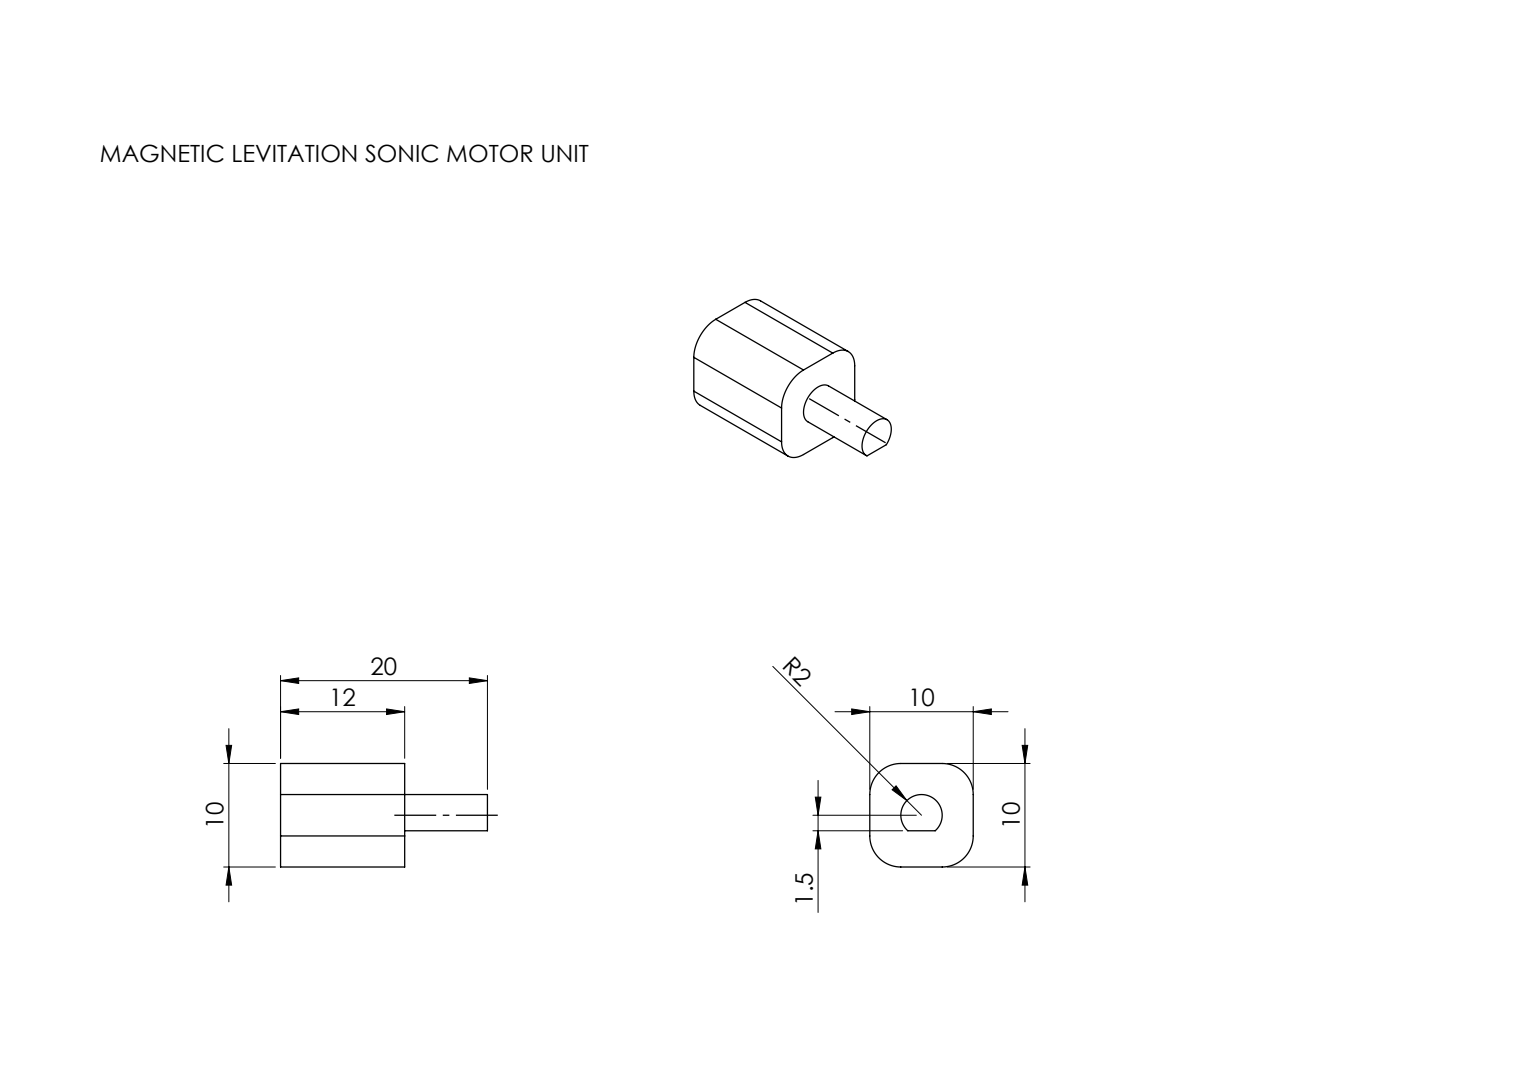
ISO-10303-21;
HEADER;
FILE_DESCRIPTION (('STEP AP214'),
    '1' );
FILE_NAME ('Magnetic Levitation Sonic Motor Unit.step',
    '2026-10-02T09:26:43',
    ( '' ),
    ( '' ),
    'SwSTEP 2.0',
    'SolidWorks 2026',
    '' );
FILE_SCHEMA (( 'AUTOMOTIVE_DESIGN' ));
ENDSEC;

DATA;
#65=DIRECTION ( 'NONE',  ( 1.000000000000000000, -0.000000000000000000, -0.000000000000000000 ) ) ;
#240=VERTEX_POINT ( 'NONE', #115266 ) ;
#450=CIRCLE ( 'NONE', #88369, 2.000000000000000000 ) ;
#508=ORIENTED_EDGE ( 'NONE', *, *, #3141, .T. ) ;
#1062=DIRECTION ( 'NONE',  ( -1.000000000000000000, 0.000000000000000000, 1.445602896647339656E-16 ) ) ;
#1136=ADVANCED_FACE ( 'NONE', ( #79104 ), #62037, .T. ) ;
#1254=CARTESIAN_POINT ( 'NONE',  ( 115.5000000000000000, 5.000000000000000000, -4.999999999999997335 ) ) ;
#1658=ORIENTED_EDGE ( 'NONE', *, *, #93470, .T. ) ;
#1663=ORIENTED_EDGE ( 'NONE', *, *, #28422, .T. ) ;
#1678=( GEOMETRIC_REPRESENTATION_CONTEXT ( 3 ) GLOBAL_UNCERTAINTY_ASSIGNED_CONTEXT ( ( #101904 ) ) GLOBAL_UNIT_ASSIGNED_CONTEXT ( ( #110801, #83298, #46567 ) ) REPRESENTATION_CONTEXT ( 'NONE', 'WORKASPACE' ) );
#1737=ORIENTED_EDGE ( 'NONE', *, *, #92849, .T. ) ;
#1889=VERTEX_POINT ( 'NONE', #49825 ) ;
#1942=AXIS2_PLACEMENT_3D ( 'NONE', #45673, #115030, #116960 ) ;
#2262=EDGE_CURVE ( 'NONE', #111941, #240, #82590, .T. ) ;
#2320=PRESENTATION_STYLE_ASSIGNMENT (( #29873 ) ) ;
#2577=DIRECTION ( 'NONE',  ( 0.000000000000000000, 0.000000000000000000, 1.000000000000000000 ) ) ;
#3141=EDGE_CURVE ( 'NONE', #1889, #72667, #15996, .T. ) ;
#3881=CARTESIAN_POINT ( 'NONE',  ( 127.5000000000000000, 2.000000000000000000, -1.999999999999998224 ) ) ;
#4111=ORIENTED_EDGE ( 'NONE', *, *, #2262, .T. ) ;
#4330=ORIENTED_EDGE ( 'NONE', *, *, #114609, .T. ) ;
#4691=SHAPE_REPRESENTATION_RELATIONSHIP ( 'NONE' , 'NONE' ,  #107120, #21197 ) ;
#5147=DIRECTION ( 'NONE',  ( 0.000000000000000000, 1.000000000000000000, -0.000000000000000000 ) ) ;
#6227=CARTESIAN_POINT ( 'NONE',  ( 115.5000000000000000, 2.000000000000000000, 5.000000000000003553 ) ) ;
#7736=ADVANCED_FACE ( 'NONE', ( #129346 ), #88749, .F. ) ;
#7761=DIRECTION ( 'NONE',  ( 7.228014483236698281E-17, 0.000000000000000000, 1.000000000000000000 ) ) ;
#8511=EDGE_CURVE ( 'NONE', #13812, #109878, #17393, .T. ) ;
#8802=CARTESIAN_POINT ( 'NONE',  ( 127.5000000000000000, -5.000000000000000000, -1.999999999999998224 ) ) ;
#9052=DIRECTION ( 'NONE',  ( -1.000000000000000000, 0.000000000000000000, 1.445602896647339656E-16 ) ) ;
#9433=ADVANCED_FACE ( 'NONE', ( #129511 ), #107901, .F. ) ;
#9447=AXIS2_PLACEMENT_3D ( 'NONE', #120852, #70463, #71758 ) ;
#10014=COLOUR_RGB ( '', 0.66274510, 0.83137255, 0.94901961) ;
#10439=AXIS2_PLACEMENT_3D ( 'NONE', #63271, #42355, #31888 ) ;
#10465=ORIENTED_EDGE ( 'NONE', *, *, #101781, .T. ) ;
#10644=CARTESIAN_POINT ( 'NONE',  ( 0.000000000000000000, 0.000000000000000000, 0.000000000000000000 ) ) ;
#10665=DIRECTION ( 'NONE',  ( 0.000000000000000000, 0.000000000000000000, -1.000000000000000000 ) ) ;
#11350=CARTESIAN_POINT ( 'NONE',  ( 127.5000000000000000, 5.000000000000000000, -4.999999999999998224 ) ) ;
#11517=SURFACE_STYLE_FILL_AREA ( #60003 ) ;
#11655=CARTESIAN_POINT ( 'NONE',  ( 127.5000000000000000, 2.000000000000000000, 5.000000000000001776 ) ) ;
#11783=CARTESIAN_POINT ( 'NONE',  ( 107.5000000000000142, 0.000000000000000000, 0.000000000000000000 ) ) ;
#12150=FILL_AREA_STYLE_COLOUR ( '', #52176 ) ;
#12190=EDGE_CURVE ( 'NONE', #36385, #240, #102708, .T. ) ;
#12224=CLOSED_SHELL ( 'NONE', ( #21549, #64318, #22970, #9433, #68328, #7736, #72582, #51956, #31701, #107579, #84007, #1136, #95844, #112044, #31528 ) ) ;
#12350=ORIENTED_EDGE ( 'NONE', *, *, #109024, .T. ) ;
#13249=ORIENTED_EDGE ( 'NONE', *, *, #43912, .F. ) ;
#13516=PLANE ( 'NONE',  #10439 ) ;
#13646=ORIENTED_EDGE ( 'NONE', *, *, #65383, .F. ) ;
#13812=VERTEX_POINT ( 'NONE', #6227 ) ;
#14010=CARTESIAN_POINT ( 'NONE',  ( 107.5000000000000142, -1.500000000000000222, -1.322875655532295136 ) ) ;
#14733=CYLINDRICAL_SURFACE ( 'NONE', #101479, 3.000000000000000000 ) ;
#14758=ORIENTED_EDGE ( 'NONE', *, *, #92576, .F. ) ;
#14831=ORIENTED_EDGE ( 'NONE', *, *, #41235, .T. ) ;
#15219=AXIS2_PLACEMENT_3D ( 'NONE', #88237, #19519, #9052 ) ;
#15562=CARTESIAN_POINT ( 'NONE',  ( 127.5000000000000000, -5.000000000000000000, -4.999999999999998224 ) ) ;
#15996=LINE ( 'NONE', #36954, #101692 ) ;
#16704=EDGE_LOOP ( 'NONE', ( #22045, #13249, #50877, #119234 ) ) ;
#16723=VERTEX_POINT ( 'NONE', #56935 ) ;
#16868=PLANE ( 'NONE',  #87019 ) ;
#16927=CARTESIAN_POINT ( 'NONE',  ( 115.5000000000000000, 0.000000000000000000, 0.000000000000000000 ) ) ;
#16966=EDGE_LOOP ( 'NONE', ( #102248, #67737, #34286, #98490 ) ) ;
#17271=DIRECTION ( 'NONE',  ( -1.000000000000000000, 0.000000000000000000, 7.228014483236698281E-17 ) ) ;
#17393=LINE ( 'NONE', #118836, #123704 ) ;
#17472=ORIENTED_EDGE ( 'NONE', *, *, #123464, .T. ) ;
#18382=CARTESIAN_POINT ( 'NONE',  ( 107.5000000000000142, 0.000000000000000000, 0.000000000000000000 ) ) ;
#18525=FACE_OUTER_BOUND ( 'NONE', #48553, .T. ) ;
#19100=PRODUCT_DEFINITION_FORMATION_WITH_SPECIFIED_SOURCE ( 'ANY', '', #126727, .NOT_KNOWN. ) ;
#19272=VECTOR ( 'NONE', #69817, 1000.000000000000000 ) ;
#19404=CYLINDRICAL_SURFACE ( 'NONE', #117385, 3.000000000000000000 ) ;
#19514=DIRECTION ( 'NONE',  ( -1.445602896647339656E-16, 0.000000000000000000, -1.000000000000000000 ) ) ;
#19519=DIRECTION ( 'NONE',  ( -1.445602896647339656E-16, 0.000000000000000000, -1.000000000000000000 ) ) ;
#20065=SURFACE_SIDE_STYLE ('',( #11517 ) ) ;
#20148=VERTEX_POINT ( 'NONE', #23352 ) ;
#20366=CYLINDRICAL_SURFACE ( 'NONE', #98432, 2.000000000000000000 ) ;
#20481=DIRECTION ( 'NONE',  ( 0.000000000000000000, 0.000000000000000000, -1.000000000000000000 ) ) ;
#20860=EDGE_CURVE ( 'NONE', #36385, #26275, #450, .T. ) ;
#21028=EDGE_CURVE ( 'NONE', #67896, #36385, #79981, .T. ) ;
#21197=ADVANCED_BREP_SHAPE_REPRESENTATION ( '', ( #100344, #108296 ), #1678 ) ;
#21549=ADVANCED_FACE ( 'NONE', ( #86151 ), #54142, .T. ) ;
#22045=ORIENTED_EDGE ( 'NONE', *, *, #39691, .T. ) ;
#22970=ADVANCED_FACE ( 'NONE', ( #100521, #58040 ), #29860, .F. ) ;
#23004=EDGE_LOOP ( 'NONE', ( #124572, #104293, #39056, #89225 ) ) ;
#23108=EDGE_LOOP ( 'NONE', ( #101575, #116612, #60474, #14758 ) ) ;
#23352=CARTESIAN_POINT ( 'NONE',  ( 127.5000000000000000, 2.000000000000000000, 5.000000000000001776 ) ) ;
#23547=AXIS2_PLACEMENT_3D ( 'NONE', #11783, #67297, #64749 ) ;
#23555=DIRECTION ( 'NONE',  ( 1.000000000000000000, 0.000000000000000000, -1.445602896647339656E-16 ) ) ;
#24253=VERTEX_POINT ( 'NONE', #107794 ) ;
#24764=AXIS2_PLACEMENT_3D ( 'NONE', #3881, #62817, #2577 ) ;
#24890=VECTOR ( 'NONE', #110517, 1000.000000000000000 ) ;
#25130=LINE ( 'NONE', #14010, #32508 ) ;
#25173=ORIENTED_EDGE ( 'NONE', *, *, #93470, .F. ) ;
#25217=ORIENTED_EDGE ( 'NONE', *, *, #65829, .F. ) ;
#25508=AXIS2_PLACEMENT_3D ( 'NONE', #64162, #104097, #82537 ) ;
#25638=FILL_AREA_STYLE_COLOUR ( '', #10014 ) ;
#25827=CARTESIAN_POINT ( 'NONE',  ( 0.000000000000000000, -5.000000000000000000, 0.000000000000000000 ) ) ;
#26275=VERTEX_POINT ( 'NONE', #82124 ) ;
#26426=DIRECTION ( 'NONE',  ( 0.000000000000000000, 0.000000000000000000, -1.000000000000000000 ) ) ;
#26535=EDGE_CURVE ( 'NONE', #13812, #82111, #34603, .T. ) ;
#26613=CARTESIAN_POINT ( 'NONE',  ( 107.5000000000000142, 0.000000000000000000, 0.000000000000000000 ) ) ;
#26943=( NAMED_UNIT ( * ) SI_UNIT ( $, .STERADIAN. ) SOLID_ANGLE_UNIT ( ) );
#28422=EDGE_CURVE ( 'NONE', #82111, #56575, #83767, .T. ) ;
#28472=DIRECTION ( 'NONE',  ( 1.000000000000000000, -0.000000000000000000, -7.228014483236698281E-17 ) ) ;
#28475=DIRECTION ( 'NONE',  ( 0.000000000000000000, 0.000000000000000000, 1.000000000000000000 ) ) ;
#29256=CARTESIAN_POINT ( 'NONE',  ( 127.5000000000000000, -2.000000000000000000, 2.000000000000001776 ) ) ;
#29359=CARTESIAN_POINT ( 'NONE',  ( 2.891205793294708895E-16, 2.000000000000000000, 2.000000000000020428 ) ) ;
#29454=AXIS2_PLACEMENT_3D ( 'NONE', #25827, #95859, #33710 ) ;
#29728=CIRCLE ( 'NONE', #25508, 2.000000000000000000 ) ;
#29854=EDGE_LOOP ( 'NONE', ( #1737, #1658, #71670, #1663 ) ) ;
#29860=PLANE ( 'NONE',  #101273 ) ;
#29873=SURFACE_STYLE_USAGE ( .BOTH. , #20065 ) ;
#29890=CARTESIAN_POINT ( 'NONE',  ( 127.5000000000000000, -2.000000000000000000, 5.000000000000001776 ) ) ;
#30716=EDGE_CURVE ( 'NONE', #127948, #48914, #48562, .T. ) ;
#30808=DIRECTION ( 'NONE',  ( 0.000000000000000000, 0.000000000000000000, 1.000000000000000000 ) ) ;
#31320=DIRECTION ( 'NONE',  ( -1.000000000000000000, -0.000000000000000000, 1.445602896647339656E-16 ) ) ;
#31425=AXIS2_PLACEMENT_3D ( 'NONE', #60506, #39589, #90580 ) ;
#31528=ADVANCED_FACE ( 'NONE', ( #36513 ), #76424, .T. ) ;
#31598=ORIENTED_EDGE ( 'NONE', *, *, #32466, .T. ) ;
#31701=ADVANCED_FACE ( 'NONE', ( #34426 ), #14733, .T. ) ;
#31888=DIRECTION ( 'NONE',  ( 0.000000000000000000, -0.000000000000000000, -1.000000000000000000 ) ) ;
#32125=CIRCLE ( 'NONE', #128264, 3.000000000000000000 ) ;
#32466=EDGE_CURVE ( 'NONE', #127948, #72667, #82415, .T. ) ;
#32508=VECTOR ( 'NONE', #36260, 1000.000000000000000 ) ;
#32961=ORIENTED_EDGE ( 'NONE', *, *, #35227, .T. ) ;
#33008=ORIENTED_EDGE ( 'NONE', *, *, #77146, .T. ) ;
#33110=STYLED_ITEM ( 'NONE', ( #74118 ), #21197 ) ;
#33710=DIRECTION ( 'NONE',  ( 0.000000000000000000, -0.000000000000000000, -1.000000000000000000 ) ) ;
#34286=ORIENTED_EDGE ( 'NONE', *, *, #109024, .F. ) ;
#34426=FACE_OUTER_BOUND ( 'NONE', #104073, .T. ) ;
#34603=CIRCLE ( 'NONE', #47193, 3.000000000000000000 ) ;
#35227=EDGE_CURVE ( 'NONE', #44931, #67896, #83560, .T. ) ;
#35416=CIRCLE ( 'NONE', #70923, 3.000000000000000000 ) ;
#35523=DIRECTION ( 'NONE',  ( 0.000000000000000000, 0.000000000000000000, 1.000000000000000000 ) ) ;
#35867=DIRECTION ( 'NONE',  ( -0.000000000000000000, -0.000000000000000000, -1.000000000000000000 ) ) ;
#35956=ORIENTED_EDGE ( 'NONE', *, *, #128508, .F. ) ;
#36260=DIRECTION ( 'NONE',  ( 1.000000000000000000, -0.000000000000000000, -0.000000000000000000 ) ) ;
#36385=VERTEX_POINT ( 'NONE', #110445 ) ;
#36513=FACE_OUTER_BOUND ( 'NONE', #102155, .T. ) ;
#36519=VECTOR ( 'NONE', #95962, 1000.000000000000000 ) ;
#36954=CARTESIAN_POINT ( 'NONE',  ( 115.5000000000000000, -2.000000000000000000, -4.999999999999997335 ) ) ;
#37326=ORIENTED_EDGE ( 'NONE', *, *, #77740, .T. ) ;
#37461=DIRECTION ( 'NONE',  ( 1.000000000000000000, -0.000000000000000000, -7.228014483236698281E-17 ) ) ;
#37515=MECHANICAL_DESIGN_GEOMETRIC_PRESENTATION_REPRESENTATION('',(#91884),#56365);
#38091=CARTESIAN_POINT ( 'NONE',  ( 115.5000000000000000, 0.000000000000000000, 0.000000000000000000 ) ) ;
#38139=VECTOR ( 'NONE', #23555, 1000.000000000000000 ) ;
#38261=FACE_OUTER_BOUND ( 'NONE', #73697, .T. ) ;
#38932=VERTEX_POINT ( 'NONE', #58490 ) ;
#39056=ORIENTED_EDGE ( 'NONE', *, *, #77146, .F. ) ;
#39564=ORIENTED_EDGE ( 'NONE', *, *, #128051, .F. ) ;
#39589=DIRECTION ( 'NONE',  ( -1.000000000000000000, 0.000000000000000000, 0.000000000000000000 ) ) ;
#39677=CARTESIAN_POINT ( 'NONE',  ( 127.5000000000000000, 5.000000000000000000, -4.999999999999998224 ) ) ;
#39691=EDGE_CURVE ( 'NONE', #84059, #111941, #77154, .T. ) ;
#39853=CIRCLE ( 'NONE', #31425, 2.000000000000000000 ) ;
#40530=EDGE_CURVE ( 'NONE', #66994, #47269, #55118, .T. ) ;
#40555=LINE ( 'NONE', #100100, #75993 ) ;
#40637=DIRECTION ( 'NONE',  ( -1.000000000000000000, 0.000000000000000000, 0.000000000000000000 ) ) ;
#40674=CARTESIAN_POINT ( 'NONE',  ( 107.5000000000000142, 0.000000000000000000, 0.000000000000000000 ) ) ;
#41021=LINE ( 'NONE', #29890, #19272 ) ;
#41235=EDGE_CURVE ( 'NONE', #20148, #13812, #62065, .T. ) ;
#41481=DIRECTION ( 'NONE',  ( -0.000000000000000000, -1.000000000000000000, -0.000000000000000000 ) ) ;
#41997=ORIENTED_EDGE ( 'NONE', *, *, #73950, .F. ) ;
#42355=DIRECTION ( 'NONE',  ( 0.000000000000000000, -1.000000000000000000, 0.000000000000000000 ) ) ;
#42949=AXIS2_PLACEMENT_3D ( 'NONE', #116083, #85335, #26426 ) ;
#43239=ORIENTED_EDGE ( 'NONE', *, *, #73950, .T. ) ;
#43912=EDGE_CURVE ( 'NONE', #67896, #111941, #129483, .T. ) ;
#44175=EDGE_LOOP ( 'NONE', ( #50268, #50582, #52858, #85813 ) ) ;
#44219=VERTEX_POINT ( 'NONE', #75668 ) ;
#44322=EDGE_LOOP ( 'NONE', ( #31598, #17472, #57035, #68258, #82847, #94300, #64121, #118110 ) ) ;
#44700=APPLICATION_CONTEXT ( 'automotive_design' ) ;
#44931=VERTEX_POINT ( 'NONE', #102724 ) ;
#45308=DIRECTION ( 'NONE',  ( 0.000000000000000000, 0.000000000000000000, 1.000000000000000000 ) ) ;
#45528=VECTOR ( 'NONE', #106603, 1000.000000000000000 ) ;
#45673=CARTESIAN_POINT ( 'NONE',  ( 115.5000000000000000, 2.000000000000000000, -1.999999999999997335 ) ) ;
#46357=CARTESIAN_POINT ( 'NONE',  ( 107.5000000000000142, -1.500000000000000222, -1.322875655532295136 ) ) ;
#46394=FACE_OUTER_BOUND ( 'NONE', #78387, .T. ) ;
#46567=( NAMED_UNIT ( * ) SI_UNIT ( $, .STERADIAN. ) SOLID_ANGLE_UNIT ( ) );
#47193=AXIS2_PLACEMENT_3D ( 'NONE', #51245, #58485, #20481 ) ;
#47269=VERTEX_POINT ( 'NONE', #98818 ) ;
#47614=ORIENTED_EDGE ( 'NONE', *, *, #88513, .T. ) ;
#47723=PRODUCT_CONTEXT ( 'NONE', #44700, 'mechanical' ) ;
#48220=CARTESIAN_POINT ( 'NONE',  ( 107.5000000000000142, -1.500000000000000222, 1.322875655532295136 ) ) ;
#48342=CARTESIAN_POINT ( 'NONE',  ( -1.445602896647332014E-16, 2.000000000000000000, -1.999999999999989120 ) ) ;
#48553=EDGE_LOOP ( 'NONE', ( #113735, #121629, #81596, #4111 ) ) ;
#48562=LINE ( 'NONE', #127758, #128709 ) ;
#48838=DIRECTION ( 'NONE',  ( 7.228014483236698281E-17, -0.000000000000000000, 1.000000000000000000 ) ) ;
#48914=VERTEX_POINT ( 'NONE', #62318 ) ;
#49825=CARTESIAN_POINT ( 'NONE',  ( 127.5000000000000000, -2.000000000000000000, -4.999999999999998224 ) ) ;
#50174=( NAMED_UNIT ( * ) SI_UNIT ( $, .STERADIAN. ) SOLID_ANGLE_UNIT ( ) );
#50268=ORIENTED_EDGE ( 'NONE', *, *, #20860, .F. ) ;
#50582=ORIENTED_EDGE ( 'NONE', *, *, #12190, .T. ) ;
#50877=ORIENTED_EDGE ( 'NONE', *, *, #35227, .F. ) ;
#51245=CARTESIAN_POINT ( 'NONE',  ( 115.5000000000000000, 2.000000000000000000, 2.000000000000003553 ) ) ;
#51462=( NAMED_UNIT ( * ) PLANE_ANGLE_UNIT ( ) SI_UNIT ( $, .RADIAN. ) );
#51956=ADVANCED_FACE ( 'NONE', ( #95218 ), #74930, .T. ) ;
#52176=COLOUR_RGB ( '', 0.66274510, 0.83137255, 0.94901961) ;
#52292=DIRECTION ( 'NONE',  ( -0.000000000000000000, -1.000000000000000000, -0.000000000000000000 ) ) ;
#52711=ORIENTED_EDGE ( 'NONE', *, *, #123234, .F. ) ;
#52858=ORIENTED_EDGE ( 'NONE', *, *, #65829, .T. ) ;
#53841=ORIENTED_EDGE ( 'NONE', *, *, #3141, .F. ) ;
#54040=DIRECTION ( 'NONE',  ( -0.000000000000000000, -0.000000000000000000, -1.000000000000000000 ) ) ;
#54142=CYLINDRICAL_SURFACE ( 'NONE', #109418, 2.000000000000000000 ) ;
#54460=SURFACE_STYLE_FILL_AREA ( #93751 ) ;
#54663=LINE ( 'NONE', #94589, #102805 ) ;
#55118=LINE ( 'NONE', #95046, #70980 ) ;
#56365=( GEOMETRIC_REPRESENTATION_CONTEXT ( 3 ) GLOBAL_UNCERTAINTY_ASSIGNED_CONTEXT ( ( #64969 ) ) GLOBAL_UNIT_ASSIGNED_CONTEXT ( ( #129393, #51462, #50174 ) ) REPRESENTATION_CONTEXT ( 'NONE', 'WORKASPACE' ) );
#56575=VERTEX_POINT ( 'NONE', #111105 ) ;
#56935=CARTESIAN_POINT ( 'NONE',  ( 115.5000000000000000, 5.000000000000000000, -1.999999999999997335 ) ) ;
#57035=ORIENTED_EDGE ( 'NONE', *, *, #40530, .T. ) ;
#57402=EDGE_CURVE ( 'NONE', #47269, #109878, #119636, .T. ) ;
#57519=VERTEX_POINT ( 'NONE', #83315 ) ;
#57656=AXIS2_PLACEMENT_3D ( 'NONE', #116793, #127917, #78184 ) ;
#58040=FACE_BOUND ( 'NONE', #83926, .T. ) ;
#58082=APPLICATION_CONTEXT ( 'automotive_design' ) ;
#58410=CIRCLE ( 'NONE', #1942, 3.000000000000000000 ) ;
#58485=DIRECTION ( 'NONE',  ( -1.000000000000000000, -0.000000000000000000, -0.000000000000000000 ) ) ;
#58490=CARTESIAN_POINT ( 'NONE',  ( 127.5000000000000000, -5.000000000000000000, -1.999999999999998224 ) ) ;
#58782=CARTESIAN_POINT ( 'NONE',  ( 107.5000000000000142, -1.500000000000000222, 1.322875655532295136 ) ) ;
#59406=VECTOR ( 'NONE', #71803, 1000.000000000000000 ) ;
#59424=VECTOR ( 'NONE', #100774, 1000.000000000000000 ) ;
#59971=VERTEX_POINT ( 'NONE', #128145 ) ;
#60003=FILL_AREA_STYLE ('',( #12150 ) ) ;
#60474=ORIENTED_EDGE ( 'NONE', *, *, #79692, .F. ) ;
#60506=CARTESIAN_POINT ( 'NONE',  ( 107.5000000000000142, 0.000000000000000000, 0.000000000000000000 ) ) ;
#61512=ORIENTED_EDGE ( 'NONE', *, *, #104934, .F. ) ;
#61821=VECTOR ( 'NONE', #98684, 1000.000000000000000 ) ;
#61837=LINE ( 'NONE', #63761, #109217 ) ;
#62037=CYLINDRICAL_SURFACE ( 'NONE', #76412, 3.000000000000000000 ) ;
#62065=LINE ( 'NONE', #11655, #88443 ) ;
#62128=AXIS2_PLACEMENT_3D ( 'NONE', #48342, #126261, #7761 ) ;
#62318=CARTESIAN_POINT ( 'NONE',  ( 127.5000000000000000, 2.000000000000000000, -4.999999999999998224 ) ) ;
#62595=CARTESIAN_POINT ( 'NONE',  ( 127.5000000000000000, 2.000000000000000000, 2.000000000000001776 ) ) ;
#62817=DIRECTION ( 'NONE',  ( 1.000000000000000000, -0.000000000000000000, -0.000000000000000000 ) ) ;
#62842=CARTESIAN_POINT ( 'NONE',  ( 2.891205793294708895E-16, 5.000000000000000000, 2.000000000000020428 ) ) ;
#63213=AXIS2_PLACEMENT_3D ( 'NONE', #120008, #121293, #10665 ) ;
#63271=CARTESIAN_POINT ( 'NONE',  ( 0.000000000000000000, 5.000000000000000000, 0.000000000000000000 ) ) ;
#63761=CARTESIAN_POINT ( 'NONE',  ( 107.5000000000000142, 0.000000000000000000, -2.000000000000000000 ) ) ;
#64121=ORIENTED_EDGE ( 'NONE', *, *, #99922, .F. ) ;
#64162=CARTESIAN_POINT ( 'NONE',  ( 115.5000000000000000, 0.000000000000000000, 0.000000000000000000 ) ) ;
#64318=ADVANCED_FACE ( 'NONE', ( #79923 ), #20366, .T. ) ;
#64749=DIRECTION ( 'NONE',  ( 0.000000000000000000, 0.000000000000000000, 1.000000000000000000 ) ) ;
#64913=ORIENTED_EDGE ( 'NONE', *, *, #123464, .F. ) ;
#64917=SURFACE_SIDE_STYLE ('',( #54460 ) ) ;
#64969=UNCERTAINTY_MEASURE_WITH_UNIT (LENGTH_MEASURE( 1.000000000000000082E-05 ), #129393, 'distance_accuracy_value', 'NONE');
#65383=EDGE_CURVE ( 'NONE', #59971, #84059, #103082, .T. ) ;
#65829=EDGE_CURVE ( 'NONE', #240, #59971, #29728, .T. ) ;
#66367=PRODUCT_DEFINITION_CONTEXT ( 'detailed design', #58082, 'design' ) ;
#66994=VERTEX_POINT ( 'NONE', #126440 ) ;
#67125=DIRECTION ( 'NONE',  ( -0.000000000000000000, -1.000000000000000000, -0.000000000000000000 ) ) ;
#67297=DIRECTION ( 'NONE',  ( -1.000000000000000000, 0.000000000000000000, 0.000000000000000000 ) ) ;
#67317=SHAPE_DEFINITION_REPRESENTATION ( #75466, #107120 ) ;
#67554=AXIS2_PLACEMENT_3D ( 'NONE', #38091, #77373, #35523 ) ;
#67647=CARTESIAN_POINT ( 'NONE',  ( 115.5000000000000000, -2.000000000000000000, -1.999999999999997335 ) ) ;
#67737=ORIENTED_EDGE ( 'NONE', *, *, #41235, .F. ) ;
#67896=VERTEX_POINT ( 'NONE', #48220 ) ;
#68258=ORIENTED_EDGE ( 'NONE', *, *, #57402, .T. ) ;
#68328=ADVANCED_FACE ( 'NONE', ( #38261 ), #107636, .F. ) ;
#69148=DIRECTION ( 'NONE',  ( 0.000000000000000000, 0.000000000000000000, 1.000000000000000000 ) ) ;
#69817=DIRECTION ( 'NONE',  ( 1.000000000000000000, 0.000000000000000000, -1.445602896647339656E-16 ) ) ;
#70463=DIRECTION ( 'NONE',  ( -1.000000000000000000, 0.000000000000000000, 0.000000000000000000 ) ) ;
#70597=CARTESIAN_POINT ( 'NONE',  ( 115.5000000000000000, 5.000000000000000000, -4.999999999999997335 ) ) ;
#70784=CARTESIAN_POINT ( 'NONE',  ( 115.5000000000000000, -5.000000000000000000, 2.000000000000003553 ) ) ;
#70923=AXIS2_PLACEMENT_3D ( 'NONE', #67647, #85363, #106293 ) ;
#70980=VECTOR ( 'NONE', #45308, 1000.000000000000000 ) ;
#71273=EDGE_LOOP ( 'NONE', ( #47614, #508, #111022, #126467 ) ) ;
#71670=ORIENTED_EDGE ( 'NONE', *, *, #99922, .T. ) ;
#71758=DIRECTION ( 'NONE',  ( 0.000000000000000000, 0.000000000000000000, 1.000000000000000000 ) ) ;
#71803=DIRECTION ( 'NONE',  ( 0.000000000000000000, 0.000000000000000000, 1.000000000000000000 ) ) ;
#72582=ADVANCED_FACE ( 'NONE', ( #92077 ), #13516, .F. ) ;
#72667=VERTEX_POINT ( 'NONE', #105781 ) ;
#72927=DIRECTION ( 'NONE',  ( 1.000000000000000000, -0.000000000000000000, -0.000000000000000000 ) ) ;
#73671=DIRECTION ( 'NONE',  ( 1.000000000000000000, 0.000000000000000000, -7.228014483236698281E-17 ) ) ;
#73697=EDGE_LOOP ( 'NONE', ( #33008, #37326, #75098, #43239, #105796, #12350, #81051, #92821 ) ) ;
#73950=EDGE_CURVE ( 'NONE', #48914, #57519, #79058, .T. ) ;
#74118=PRESENTATION_STYLE_ASSIGNMENT (( #104208 ) ) ;
#74930=PLANE ( 'NONE',  #29454 ) ;
#74973=CARTESIAN_POINT ( 'NONE',  ( 127.5000000000000000, -2.000000000000000000, -1.999999999999998224 ) ) ;
#75098=ORIENTED_EDGE ( 'NONE', *, *, #88513, .F. ) ;
#75466=PRODUCT_DEFINITION_SHAPE ( 'NONE', 'NONE',  #98771 ) ;
#75615=VECTOR ( 'NONE', #41481, 1000.000000000000000 ) ;
#75662=CARTESIAN_POINT ( 'NONE',  ( 127.5000000000000000, 5.000000000000000000, 5.000000000000001776 ) ) ;
#75668=CARTESIAN_POINT ( 'NONE',  ( 127.5000000000000000, -5.000000000000000000, 2.000000000000001776 ) ) ;
#75686=DIRECTION ( 'NONE',  ( 0.000000000000000000, 0.000000000000000000, 1.000000000000000000 ) ) ;
#75696=DIRECTION ( 'NONE',  ( 0.000000000000000000, 0.000000000000000000, -1.000000000000000000 ) ) ;
#75857=CARTESIAN_POINT ( 'NONE',  ( 115.5000000000000000, -1.500000000000000222, -1.322875655532295136 ) ) ;
#75993=VECTOR ( 'NONE', #79804, 1000.000000000000000 ) ;
#76371=EDGE_CURVE ( 'NONE', #44219, #47269, #119888, .T. ) ;
#76412=AXIS2_PLACEMENT_3D ( 'NONE', #29359, #99383, #19514 ) ;
#76424=PLANE ( 'NONE',  #9447 ) ;
#76922=CARTESIAN_POINT ( 'NONE',  ( 127.5000000000000000, -2.000000000000000000, -1.999999999999998224 ) ) ;
#77146=EDGE_CURVE ( 'NONE', #44219, #38932, #106528, .T. ) ;
#77154=LINE ( 'NONE', #94860, #45528 ) ;
#77373=DIRECTION ( 'NONE',  ( -1.000000000000000000, 0.000000000000000000, 0.000000000000000000 ) ) ;
#77740=EDGE_CURVE ( 'NONE', #38932, #1889, #125814, .T. ) ;
#78184=DIRECTION ( 'NONE',  ( 0.000000000000000000, 0.000000000000000000, 1.000000000000000000 ) ) ;
#78387=EDGE_LOOP ( 'NONE', ( #41997, #90187, #52711, #25173 ) ) ;
#78710=CARTESIAN_POINT ( 'NONE',  ( 115.5000000000000000, -2.000000000000000000, 5.000000000000003553 ) ) ;
#79058=CIRCLE ( 'NONE', #24764, 3.000000000000000000 ) ;
#79104=FACE_OUTER_BOUND ( 'NONE', #16966, .T. ) ;
#79604=DIRECTION ( 'NONE',  ( 0.000000000000000000, 0.000000000000000000, -1.000000000000000000 ) ) ;
#79692=EDGE_CURVE ( 'NONE', #24253, #44219, #32125, .T. ) ;
#79804=DIRECTION ( 'NONE',  ( -1.000000000000000000, 0.000000000000000000, 7.228014483236698281E-17 ) ) ;
#79923=FACE_OUTER_BOUND ( 'NONE', #120795, .T. ) ;
#79981=CIRCLE ( 'NONE', #23547, 2.000000000000000000 ) ;
#80718=DIRECTION ( 'NONE',  ( 1.000000000000000000, 0.000000000000000000, 0.000000000000000000 ) ) ;
#81051=ORIENTED_EDGE ( 'NONE', *, *, #128051, .T. ) ;
#81596=ORIENTED_EDGE ( 'NONE', *, *, #43912, .T. ) ;
#82111=VERTEX_POINT ( 'NONE', #89746 ) ;
#82124=CARTESIAN_POINT ( 'NONE',  ( 107.5000000000000142, 0.000000000000000000, -2.000000000000000000 ) ) ;
#82212=FACE_OUTER_BOUND ( 'NONE', #23108, .T. ) ;
#82415=LINE ( 'NONE', #1254, #83691 ) ;
#82537=DIRECTION ( 'NONE',  ( 0.000000000000000000, 0.000000000000000000, 1.000000000000000000 ) ) ;
#82590=CIRCLE ( 'NONE', #105665, 2.000000000000000000 ) ;
#82847=ORIENTED_EDGE ( 'NONE', *, *, #8511, .F. ) ;
#83298=( NAMED_UNIT ( * ) PLANE_ANGLE_UNIT ( ) SI_UNIT ( $, .RADIAN. ) );
#83315=CARTESIAN_POINT ( 'NONE',  ( 127.5000000000000000, 5.000000000000000000, -1.999999999999998224 ) ) ;
#83560=LINE ( 'NONE', #101902, #59406 ) ;
#83623=ORIENTED_EDGE ( 'NONE', *, *, #65383, .T. ) ;
#83691=VECTOR ( 'NONE', #52292, 1000.000000000000000 ) ;
#83767=LINE ( 'NONE', #62842, #38139 ) ;
#83926=EDGE_LOOP ( 'NONE', ( #85902, #127427, #13646, #25217 ) ) ;
#84007=ADVANCED_FACE ( 'NONE', ( #46394 ), #108552, .T. ) ;
#84059=VERTEX_POINT ( 'NONE', #75857 ) ;
#84361=CARTESIAN_POINT ( 'NONE',  ( 115.5000000000000000, -1.500000000000000222, 1.322875655532295136 ) ) ;
#84874=CARTESIAN_POINT ( 'NONE',  ( 127.5000000000000000, -2.000000000000000000, 2.000000000000001776 ) ) ;
#85335=DIRECTION ( 'NONE',  ( 1.000000000000000000, -0.000000000000000000, -0.000000000000000000 ) ) ;
#85363=DIRECTION ( 'NONE',  ( -1.000000000000000000, -0.000000000000000000, -0.000000000000000000 ) ) ;
#85813=ORIENTED_EDGE ( 'NONE', *, *, #114609, .F. ) ;
#85902=ORIENTED_EDGE ( 'NONE', *, *, #2262, .F. ) ;
#86095=AXIS2_PLACEMENT_3D ( 'NONE', #76922, #107674, #28475 ) ;
#86151=FACE_OUTER_BOUND ( 'NONE', #44175, .T. ) ;
#87019=AXIS2_PLACEMENT_3D ( 'NONE', #46357, #5147, #115084 ) ;
#87628=DIRECTION ( 'NONE',  ( -1.000000000000000000, 0.000000000000000000, 0.000000000000000000 ) ) ;
#87949=EDGE_LOOP ( 'NONE', ( #94799, #102039, #39564, #14831 ) ) ;
#88237=CARTESIAN_POINT ( 'NONE',  ( 127.5000000000000000, 5.000000000000000000, 5.000000000000001776 ) ) ;
#88369=AXIS2_PLACEMENT_3D ( 'NONE', #18382, #40637, #30808 ) ;
#88443=VECTOR ( 'NONE', #31320, 1000.000000000000000 ) ;
#88513=EDGE_CURVE ( 'NONE', #48914, #1889, #101015, .T. ) ;
#88749=PLANE ( 'NONE',  #116558 ) ;
#89225=ORIENTED_EDGE ( 'NONE', *, *, #76371, .T. ) ;
#89746=CARTESIAN_POINT ( 'NONE',  ( 115.5000000000000000, 5.000000000000000000, 2.000000000000003553 ) ) ;
#90187=ORIENTED_EDGE ( 'NONE', *, *, #30716, .F. ) ;
#90516=DIRECTION ( 'NONE',  ( 0.000000000000000000, 0.000000000000000000, 1.000000000000000000 ) ) ;
#90580=DIRECTION ( 'NONE',  ( 0.000000000000000000, 0.000000000000000000, 1.000000000000000000 ) ) ;
#91577=MECHANICAL_DESIGN_GEOMETRIC_PRESENTATION_REPRESENTATION('',(#33110),#129263);
#91884=STYLED_ITEM ( 'NONE', ( #2320 ), #100344 ) ;
#92017=VECTOR ( 'NONE', #108130, 1000.000000000000000 ) ;
#92077=FACE_OUTER_BOUND ( 'NONE', #29854, .T. ) ;
#92385=CARTESIAN_POINT ( 'NONE',  ( 115.5000000000000000, 2.000000000000000000, -4.999999999999997335 ) ) ;
#92576=EDGE_CURVE ( 'NONE', #109878, #24253, #41021, .T. ) ;
#92821=ORIENTED_EDGE ( 'NONE', *, *, #79692, .T. ) ;
#92849=EDGE_CURVE ( 'NONE', #56575, #57519, #54663, .T. ) ;
#93470=EDGE_CURVE ( 'NONE', #57519, #16723, #40555, .T. ) ;
#93751=FILL_AREA_STYLE ('',( #25638 ) ) ;
#94065=DIRECTION ( 'NONE',  ( 1.000000000000000000, -0.000000000000000000, -0.000000000000000000 ) ) ;
#94300=ORIENTED_EDGE ( 'NONE', *, *, #26535, .T. ) ;
#94589=CARTESIAN_POINT ( 'NONE',  ( 127.5000000000000000, 5.000000000000000000, -4.999999999999998224 ) ) ;
#94597=DIRECTION ( 'NONE',  ( 0.000000000000000000, 0.000000000000000000, -1.000000000000000000 ) ) ;
#94799=ORIENTED_EDGE ( 'NONE', *, *, #8511, .T. ) ;
#94825=FACE_OUTER_BOUND ( 'NONE', #16704, .T. ) ;
#94860=CARTESIAN_POINT ( 'NONE',  ( 115.5000000000000000, -1.500000000000000222, -1.322875655532295136 ) ) ;
#95046=CARTESIAN_POINT ( 'NONE',  ( 115.5000000000000000, -5.000000000000000000, -4.999999999999997335 ) ) ;
#95162=CYLINDRICAL_SURFACE ( 'NONE', #42949, 2.000000000000000000 ) ;
#95218=FACE_OUTER_BOUND ( 'NONE', #23004, .T. ) ;
#95844=ADVANCED_FACE ( 'NONE', ( #18525 ), #95162, .T. ) ;
#95859=DIRECTION ( 'NONE',  ( 0.000000000000000000, -1.000000000000000000, 0.000000000000000000 ) ) ;
#95962=DIRECTION ( 'NONE',  ( -0.000000000000000000, -1.000000000000000000, -0.000000000000000000 ) ) ;
#96881=VECTOR ( 'NONE', #28472, 1000.000000000000000 ) ;
#98432=AXIS2_PLACEMENT_3D ( 'NONE', #40674, #65, #110665 ) ;
#98490=ORIENTED_EDGE ( 'NONE', *, *, #28422, .F. ) ;
#98684=DIRECTION ( 'NONE',  ( 1.000000000000000000, -0.000000000000000000, -0.000000000000000000 ) ) ;
#98736=DIRECTION ( 'NONE',  ( 0.000000000000000000, 0.000000000000000000, 1.000000000000000000 ) ) ;
#98771=PRODUCT_DEFINITION ( 'UNKNOWN', '', #19100, #66367 ) ;
#98818=CARTESIAN_POINT ( 'NONE',  ( 115.5000000000000000, -5.000000000000000000, 2.000000000000003553 ) ) ;
#99383=DIRECTION ( 'NONE',  ( 1.000000000000000000, 0.000000000000000000, -1.445602896647339656E-16 ) ) ;
#99922=EDGE_CURVE ( 'NONE', #16723, #82111, #101995, .T. ) ;
#100100=CARTESIAN_POINT ( 'NONE',  ( -1.445602896647332014E-16, 5.000000000000000000, -1.999999999999989120 ) ) ;
#100344=MANIFOLD_SOLID_BREP ( 'Boss-Extrude2', #12224 ) ;
#100521=FACE_OUTER_BOUND ( 'NONE', #44322, .T. ) ;
#100774=DIRECTION ( 'NONE',  ( 1.000000000000000000, -0.000000000000000000, -0.000000000000000000 ) ) ;
#101015=LINE ( 'NONE', #11350, #75615 ) ;
#101222=DIRECTION ( 'NONE',  ( 0.000000000000000000, 0.000000000000000000, 1.000000000000000000 ) ) ;
#101273=AXIS2_PLACEMENT_3D ( 'NONE', #109038, #127418, #79604 ) ;
#101479=AXIS2_PLACEMENT_3D ( 'NONE', #74973, #73671, #94597 ) ;
#101575=ORIENTED_EDGE ( 'NONE', *, *, #57402, .F. ) ;
#101692=VECTOR ( 'NONE', #17271, 1000.000000000000000 ) ;
#101781=EDGE_CURVE ( 'NONE', #26275, #44931, #39853, .T. ) ;
#101902=CARTESIAN_POINT ( 'NONE',  ( 107.5000000000000142, -1.500000000000000222, -1.322875655532295136 ) ) ;
#101904=UNCERTAINTY_MEASURE_WITH_UNIT (LENGTH_MEASURE( 1.000000000000000082E-05 ), #110801, 'distance_accuracy_value', 'NONE');
#101995=LINE ( 'NONE', #70597, #24890 ) ;
#102039=ORIENTED_EDGE ( 'NONE', *, *, #92576, .T. ) ;
#102155=EDGE_LOOP ( 'NONE', ( #118710, #127254, #10465, #32961 ) ) ;
#102248=ORIENTED_EDGE ( 'NONE', *, *, #26535, .F. ) ;
#102708=LINE ( 'NONE', #111235, #59424 ) ;
#102724=CARTESIAN_POINT ( 'NONE',  ( 107.5000000000000142, -1.500000000000000222, -1.322875655532295136 ) ) ;
#102805=VECTOR ( 'NONE', #54040, 1000.000000000000000 ) ;
#103082=CIRCLE ( 'NONE', #67554, 2.000000000000000000 ) ;
#104073=EDGE_LOOP ( 'NONE', ( #118450, #61512, #64913, #53841 ) ) ;
#104097=DIRECTION ( 'NONE',  ( -1.000000000000000000, 0.000000000000000000, 0.000000000000000000 ) ) ;
#104208=SURFACE_STYLE_USAGE ( .BOTH. , #64917 ) ;
#104293=ORIENTED_EDGE ( 'NONE', *, *, #104934, .T. ) ;
#104838=( LENGTH_UNIT ( ) NAMED_UNIT ( * ) SI_UNIT ( .MILLI., .METRE. ) );
#104934=EDGE_CURVE ( 'NONE', #66994, #38932, #118123, .T. ) ;
#105665=AXIS2_PLACEMENT_3D ( 'NONE', #16927, #87628, #98736 ) ;
#105781=CARTESIAN_POINT ( 'NONE',  ( 115.5000000000000000, -2.000000000000000000, -4.999999999999997335 ) ) ;
#105796=ORIENTED_EDGE ( 'NONE', *, *, #92849, .F. ) ;
#106293=DIRECTION ( 'NONE',  ( 0.000000000000000000, 0.000000000000000000, -1.000000000000000000 ) ) ;
#106528=LINE ( 'NONE', #15562, #125712 ) ;
#106603=DIRECTION ( 'NONE',  ( 0.000000000000000000, 0.000000000000000000, 1.000000000000000000 ) ) ;
#107120=SHAPE_REPRESENTATION ( 'Magnetic Levitation Sonic Motor Unit', ( #108296 ), #1678 ) ;
#107579=ADVANCED_FACE ( 'NONE', ( #82212 ), #19404, .T. ) ;
#107636=PLANE ( 'NONE',  #57656 ) ;
#107674=DIRECTION ( 'NONE',  ( 1.000000000000000000, -0.000000000000000000, -0.000000000000000000 ) ) ;
#107794=CARTESIAN_POINT ( 'NONE',  ( 127.5000000000000000, -2.000000000000000000, 5.000000000000001776 ) ) ;
#107901=PLANE ( 'NONE',  #15219 ) ;
#108130=DIRECTION ( 'NONE',  ( -1.000000000000000000, -0.000000000000000000, 1.445602896647339656E-16 ) ) ;
#108296=AXIS2_PLACEMENT_3D ( 'NONE', #10644, #90516, #80718 ) ;
#108552=CYLINDRICAL_SURFACE ( 'NONE', #62128, 3.000000000000000000 ) ;
#109024=EDGE_CURVE ( 'NONE', #56575, #20148, #113675, .T. ) ;
#109038=CARTESIAN_POINT ( 'NONE',  ( 115.5000000000000000, 5.000000000000000000, -4.999999999999997335 ) ) ;
#109217=VECTOR ( 'NONE', #72927, 1000.000000000000000 ) ;
#109354=ORIENTED_EDGE ( 'NONE', *, *, #101781, .F. ) ;
#109418=AXIS2_PLACEMENT_3D ( 'NONE', #26613, #94065, #75696 ) ;
#109878=VERTEX_POINT ( 'NONE', #78710 ) ;
#110445=CARTESIAN_POINT ( 'NONE',  ( 107.5000000000000142, 2.449293598294706414E-16, 2.000000000000000000 ) ) ;
#110517=DIRECTION ( 'NONE',  ( 0.000000000000000000, 0.000000000000000000, 1.000000000000000000 ) ) ;
#110665=DIRECTION ( 'NONE',  ( 0.000000000000000000, 0.000000000000000000, -1.000000000000000000 ) ) ;
#110801=( LENGTH_UNIT ( ) NAMED_UNIT ( * ) SI_UNIT ( .MILLI., .METRE. ) );
#111022=ORIENTED_EDGE ( 'NONE', *, *, #32466, .F. ) ;
#111105=CARTESIAN_POINT ( 'NONE',  ( 127.5000000000000000, 5.000000000000000000, 2.000000000000001776 ) ) ;
#111235=CARTESIAN_POINT ( 'NONE',  ( 107.5000000000000142, 2.449293598294706414E-16, 2.000000000000000000 ) ) ;
#111941=VERTEX_POINT ( 'NONE', #84361 ) ;
#112044=ADVANCED_FACE ( 'NONE', ( #94825 ), #16868, .F. ) ;
#112372=UNCERTAINTY_MEASURE_WITH_UNIT (LENGTH_MEASURE( 1.000000000000000082E-05 ), #104838, 'distance_accuracy_value', 'NONE');
#113675=CIRCLE ( 'NONE', #128363, 3.000000000000000000 ) ;
#113735=ORIENTED_EDGE ( 'NONE', *, *, #12190, .F. ) ;
#114609=EDGE_CURVE ( 'NONE', #26275, #59971, #61837, .T. ) ;
#115030=DIRECTION ( 'NONE',  ( -1.000000000000000000, -0.000000000000000000, -0.000000000000000000 ) ) ;
#115084=DIRECTION ( 'NONE',  ( 0.000000000000000000, 0.000000000000000000, 1.000000000000000000 ) ) ;
#115266=CARTESIAN_POINT ( 'NONE',  ( 115.5000000000000000, 2.449293598294706414E-16, 2.000000000000000000 ) ) ;
#116083=CARTESIAN_POINT ( 'NONE',  ( 107.5000000000000142, 0.000000000000000000, 0.000000000000000000 ) ) ;
#116558=AXIS2_PLACEMENT_3D ( 'NONE', #39677, #48838, #119485 ) ;
#116597=( NAMED_UNIT ( * ) PLANE_ANGLE_UNIT ( ) SI_UNIT ( $, .RADIAN. ) );
#116612=ORIENTED_EDGE ( 'NONE', *, *, #76371, .F. ) ;
#116793=CARTESIAN_POINT ( 'NONE',  ( 127.5000000000000000, 5.000000000000000000, -4.999999999999998224 ) ) ;
#116960=DIRECTION ( 'NONE',  ( 0.000000000000000000, 0.000000000000000000, -1.000000000000000000 ) ) ;
#117385=AXIS2_PLACEMENT_3D ( 'NONE', #29256, #1062, #69148 ) ;
#118110=ORIENTED_EDGE ( 'NONE', *, *, #123234, .T. ) ;
#118123=LINE ( 'NONE', #8802, #96881 ) ;
#118450=ORIENTED_EDGE ( 'NONE', *, *, #77740, .F. ) ;
#118710=ORIENTED_EDGE ( 'NONE', *, *, #21028, .T. ) ;
#118836=CARTESIAN_POINT ( 'NONE',  ( 115.5000000000000000, 5.000000000000000000, 5.000000000000003553 ) ) ;
#119234=ORIENTED_EDGE ( 'NONE', *, *, #128508, .T. ) ;
#119485=DIRECTION ( 'NONE',  ( 1.000000000000000000, 0.000000000000000000, -7.228014483236698281E-17 ) ) ;
#119554=DIRECTION ( 'NONE',  ( 1.000000000000000000, -0.000000000000000000, -0.000000000000000000 ) ) ;
#119636=CIRCLE ( 'NONE', #63213, 3.000000000000000000 ) ;
#119888=LINE ( 'NONE', #70784, #92017 ) ;
#120008=CARTESIAN_POINT ( 'NONE',  ( 115.5000000000000000, -2.000000000000000000, 2.000000000000003553 ) ) ;
#120795=EDGE_LOOP ( 'NONE', ( #109354, #4330, #83623, #35956 ) ) ;
#120852=CARTESIAN_POINT ( 'NONE',  ( 107.5000000000000142, 0.000000000000000000, 0.000000000000000000 ) ) ;
#121293=DIRECTION ( 'NONE',  ( -1.000000000000000000, -0.000000000000000000, -0.000000000000000000 ) ) ;
#121629=ORIENTED_EDGE ( 'NONE', *, *, #21028, .F. ) ;
#123234=EDGE_CURVE ( 'NONE', #16723, #127948, #58410, .T. ) ;
#123464=EDGE_CURVE ( 'NONE', #72667, #66994, #35416, .T. ) ;
#123704=VECTOR ( 'NONE', #67125, 1000.000000000000000 ) ;
#124572=ORIENTED_EDGE ( 'NONE', *, *, #40530, .F. ) ;
#124784=LINE ( 'NONE', #75662, #36519 ) ;
#124810=DIRECTION ( 'NONE',  ( 1.000000000000000000, -0.000000000000000000, -0.000000000000000000 ) ) ;
#125712=VECTOR ( 'NONE', #35867, 1000.000000000000000 ) ;
#125814=CIRCLE ( 'NONE', #86095, 3.000000000000000000 ) ;
#126261=DIRECTION ( 'NONE',  ( -1.000000000000000000, 0.000000000000000000, 7.228014483236698281E-17 ) ) ;
#126440=CARTESIAN_POINT ( 'NONE',  ( 115.5000000000000000, -5.000000000000000000, -1.999999999999997335 ) ) ;
#126467=ORIENTED_EDGE ( 'NONE', *, *, #30716, .T. ) ;
#126727=PRODUCT ( 'Magnetic Levitation Sonic Motor Unit', 'Magnetic Levitation Sonic Motor Unit', '', ( #47723 ) ) ;
#127254=ORIENTED_EDGE ( 'NONE', *, *, #20860, .T. ) ;
#127418=DIRECTION ( 'NONE',  ( 1.000000000000000000, 0.000000000000000000, 0.000000000000000000 ) ) ;
#127427=ORIENTED_EDGE ( 'NONE', *, *, #39691, .F. ) ;
#127758=CARTESIAN_POINT ( 'NONE',  ( 127.5000000000000000, 2.000000000000000000, -4.999999999999998224 ) ) ;
#127917=DIRECTION ( 'NONE',  ( -1.000000000000000000, 0.000000000000000000, 0.000000000000000000 ) ) ;
#127948=VERTEX_POINT ( 'NONE', #92385 ) ;
#128051=EDGE_CURVE ( 'NONE', #20148, #24253, #124784, .T. ) ;
#128145=CARTESIAN_POINT ( 'NONE',  ( 115.5000000000000000, 0.000000000000000000, -2.000000000000000000 ) ) ;
#128264=AXIS2_PLACEMENT_3D ( 'NONE', #84874, #124810, #75686 ) ;
#128363=AXIS2_PLACEMENT_3D ( 'NONE', #62595, #119554, #101222 ) ;
#128508=EDGE_CURVE ( 'NONE', #44931, #84059, #25130, .T. ) ;
#128709=VECTOR ( 'NONE', #37461, 1000.000000000000000 ) ;
#129263=( GEOMETRIC_REPRESENTATION_CONTEXT ( 3 ) GLOBAL_UNCERTAINTY_ASSIGNED_CONTEXT ( ( #112372 ) ) GLOBAL_UNIT_ASSIGNED_CONTEXT ( ( #104838, #116597, #26943 ) ) REPRESENTATION_CONTEXT ( 'NONE', 'WORKASPACE' ) );
#129346=FACE_OUTER_BOUND ( 'NONE', #71273, .T. ) ;
#129393=( LENGTH_UNIT ( ) NAMED_UNIT ( * ) SI_UNIT ( .MILLI., .METRE. ) );
#129483=LINE ( 'NONE', #58782, #61821 ) ;
#129511=FACE_OUTER_BOUND ( 'NONE', #87949, .T. ) ;
ENDSEC;
END-ISO-10303-21;
